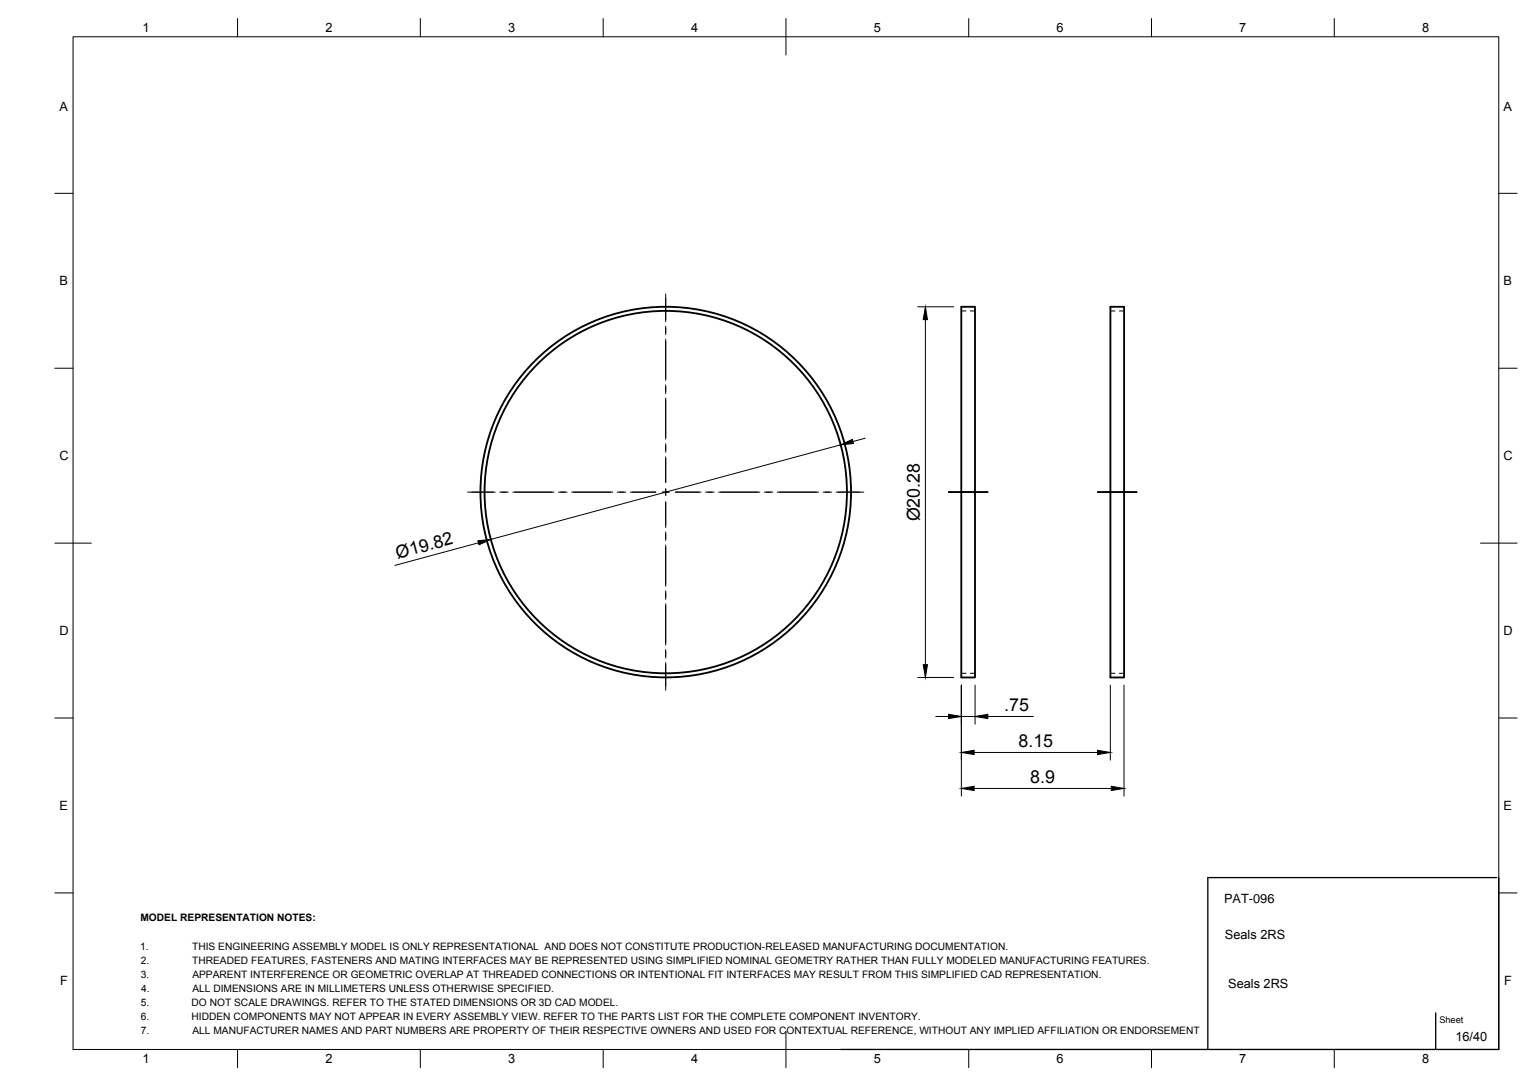
ISO-10303-21;
HEADER;
/* Generated by software containing ST-Developer
 * from STEP Tools, Inc. (www.steptools.com) 
 */

FILE_DESCRIPTION(
/* description */ ('PAT-096'),
/* implementation_level */ '2;1');

FILE_NAME(
/* name */ 'Seals 2RS.step',
/* time_stamp */ '2026-10-29T17:03:14-07:00',
/* author */ (''),
/* organization */ (''),
/* preprocessor_version */ 'ST-DEVELOPER v20.2',
/* originating_system */ 'Autodesk Translation Framework v15.17.0.0',
/* authorisation */ '');

FILE_SCHEMA (('AUTOMOTIVE_DESIGN { 1 0 10303 214 3 1 1 }'));
ENDSEC;

DATA;
#10=MECHANICAL_DESIGN_GEOMETRIC_PRESENTATION_REPRESENTATION('',(#413,#414),#10650);
#344=SHAPE_REPRESENTATION_RELATIONSHIP('SRR','None',#10805,#375);
#375=ADVANCED_BREP_SHAPE_REPRESENTATION('',(#451,#452),#10623);
#413=STYLED_ITEM('',(#11064),#451);
#414=STYLED_ITEM('',(#11064),#452);
#451=MANIFOLD_SOLID_BREP('Body1',#5547);
#452=MANIFOLD_SOLID_BREP('Body2',#5548);
#528=FACE_BOUND('',#1302,.T.);
#529=FACE_BOUND('',#1305,.T.);
#530=FACE_BOUND('',#1308,.T.);
#531=FACE_BOUND('',#1311,.T.);
#661=PLANE('',#6196);
#662=PLANE('',#6201);
#663=PLANE('',#6204);
#664=PLANE('',#6209);
#910=FACE_OUTER_BOUND('',#1301,.T.);
#911=FACE_OUTER_BOUND('',#1303,.T.);
#912=FACE_OUTER_BOUND('',#1304,.T.);
#913=FACE_OUTER_BOUND('',#1306,.T.);
#914=FACE_OUTER_BOUND('',#1307,.T.);
#915=FACE_OUTER_BOUND('',#1309,.T.);
#916=FACE_OUTER_BOUND('',#1310,.T.);
#917=FACE_OUTER_BOUND('',#1312,.T.);
#1301=EDGE_LOOP('',(#4231));
#1302=EDGE_LOOP('',(#4232));
#1303=EDGE_LOOP('',(#4233,#4234,#4235,#4236));
#1304=EDGE_LOOP('',(#4237));
#1305=EDGE_LOOP('',(#4238));
#1306=EDGE_LOOP('',(#4239,#4240,#4241,#4242));
#1307=EDGE_LOOP('',(#4243));
#1308=EDGE_LOOP('',(#4244));
#1309=EDGE_LOOP('',(#4245,#4246,#4247,#4248));
#1310=EDGE_LOOP('',(#4249));
#1311=EDGE_LOOP('',(#4250));
#1312=EDGE_LOOP('',(#4251,#4252,#4253,#4254));
#1688=LINE('',#9497,#2017);
#1689=LINE('',#9502,#2018);
#1690=LINE('',#9511,#2019);
#1691=LINE('',#9516,#2020);
#2017=VECTOR('',#7330,1.013815);
#2018=VECTOR('',#7337,0.991185);
#2019=VECTOR('',#7348,1.013815);
#2020=VECTOR('',#7355,0.991185);
#2408=CIRCLE('',#6197,1.013815);
#2409=CIRCLE('',#6198,0.991185);
#2410=CIRCLE('',#6200,1.013815);
#2411=CIRCLE('',#6202,0.991185);
#2412=CIRCLE('',#6205,1.013815);
#2413=CIRCLE('',#6206,0.991185);
#2414=CIRCLE('',#6208,1.013815);
#2415=CIRCLE('',#6210,0.991185);
#2759=VERTEX_POINT('',#9490);
#2760=VERTEX_POINT('',#9492);
#2761=VERTEX_POINT('',#9495);
#2762=VERTEX_POINT('',#9499);
#2763=VERTEX_POINT('',#9504);
#2764=VERTEX_POINT('',#9506);
#2765=VERTEX_POINT('',#9509);
#2766=VERTEX_POINT('',#9513);
#3294=EDGE_CURVE('',#2759,#2759,#2408,.T.);
#3295=EDGE_CURVE('',#2760,#2760,#2409,.T.);
#3296=EDGE_CURVE('',#2761,#2761,#2410,.T.);
#3297=EDGE_CURVE('',#2761,#2759,#1688,.T.);
#3298=EDGE_CURVE('',#2762,#2762,#2411,.T.);
#3299=EDGE_CURVE('',#2762,#2760,#1689,.T.);
#3300=EDGE_CURVE('',#2763,#2763,#2412,.T.);
#3301=EDGE_CURVE('',#2764,#2764,#2413,.T.);
#3302=EDGE_CURVE('',#2765,#2765,#2414,.T.);
#3303=EDGE_CURVE('',#2765,#2763,#1690,.T.);
#3304=EDGE_CURVE('',#2766,#2766,#2415,.T.);
#3305=EDGE_CURVE('',#2766,#2764,#1691,.T.);
#4231=ORIENTED_EDGE('',*,*,#3294,.F.);
#4232=ORIENTED_EDGE('',*,*,#3295,.T.);
#4233=ORIENTED_EDGE('',*,*,#3296,.F.);
#4234=ORIENTED_EDGE('',*,*,#3297,.T.);
#4235=ORIENTED_EDGE('',*,*,#3294,.T.);
#4236=ORIENTED_EDGE('',*,*,#3297,.F.);
#4237=ORIENTED_EDGE('',*,*,#3296,.T.);
#4238=ORIENTED_EDGE('',*,*,#3298,.F.);
#4239=ORIENTED_EDGE('',*,*,#3298,.T.);
#4240=ORIENTED_EDGE('',*,*,#3299,.T.);
#4241=ORIENTED_EDGE('',*,*,#3295,.F.);
#4242=ORIENTED_EDGE('',*,*,#3299,.F.);
#4243=ORIENTED_EDGE('',*,*,#3300,.F.);
#4244=ORIENTED_EDGE('',*,*,#3301,.T.);
#4245=ORIENTED_EDGE('',*,*,#3302,.F.);
#4246=ORIENTED_EDGE('',*,*,#3303,.T.);
#4247=ORIENTED_EDGE('',*,*,#3300,.T.);
#4248=ORIENTED_EDGE('',*,*,#3303,.F.);
#4249=ORIENTED_EDGE('',*,*,#3302,.T.);
#4250=ORIENTED_EDGE('',*,*,#3304,.F.);
#4251=ORIENTED_EDGE('',*,*,#3304,.T.);
#4252=ORIENTED_EDGE('',*,*,#3305,.T.);
#4253=ORIENTED_EDGE('',*,*,#3301,.F.);
#4254=ORIENTED_EDGE('',*,*,#3305,.F.);
#5119=CYLINDRICAL_SURFACE('',#6199,1.013815);
#5120=CYLINDRICAL_SURFACE('',#6203,0.991185);
#5121=CYLINDRICAL_SURFACE('',#6207,1.013815);
#5122=CYLINDRICAL_SURFACE('',#6211,0.991185);
#5315=ADVANCED_FACE('',(#910,#528),#661,.T.);
#5316=ADVANCED_FACE('',(#911),#5119,.T.);
#5317=ADVANCED_FACE('',(#912,#529),#662,.T.);
#5318=ADVANCED_FACE('',(#913),#5120,.F.);
#5319=ADVANCED_FACE('',(#914,#530),#663,.T.);
#5320=ADVANCED_FACE('',(#915),#5121,.T.);
#5321=ADVANCED_FACE('',(#916,#531),#664,.T.);
#5322=ADVANCED_FACE('',(#917),#5122,.F.);
#5547=CLOSED_SHELL('',(#5315,#5316,#5317,#5318));
#5548=CLOSED_SHELL('',(#5319,#5320,#5321,#5322));
#6195=AXIS2_PLACEMENT_3D('',#9488,#7318,#7319);
#6196=AXIS2_PLACEMENT_3D('',#9489,#7320,#7321);
#6197=AXIS2_PLACEMENT_3D('',#9491,#7322,#7323);
#6198=AXIS2_PLACEMENT_3D('',#9493,#7324,#7325);
#6199=AXIS2_PLACEMENT_3D('',#9494,#7326,#7327);
#6200=AXIS2_PLACEMENT_3D('',#9496,#7328,#7329);
#6201=AXIS2_PLACEMENT_3D('',#9498,#7331,#7332);
#6202=AXIS2_PLACEMENT_3D('',#9500,#7333,#7334);
#6203=AXIS2_PLACEMENT_3D('',#9501,#7335,#7336);
#6204=AXIS2_PLACEMENT_3D('',#9503,#7338,#7339);
#6205=AXIS2_PLACEMENT_3D('',#9505,#7340,#7341);
#6206=AXIS2_PLACEMENT_3D('',#9507,#7342,#7343);
#6207=AXIS2_PLACEMENT_3D('',#9508,#7344,#7345);
#6208=AXIS2_PLACEMENT_3D('',#9510,#7346,#7347);
#6209=AXIS2_PLACEMENT_3D('',#9512,#7349,#7350);
#6210=AXIS2_PLACEMENT_3D('',#9514,#7351,#7352);
#6211=AXIS2_PLACEMENT_3D('',#9515,#7353,#7354);
#7318=DIRECTION('axis',(0.,0.,1.));
#7319=DIRECTION('refdir',(1.,0.,0.));
#7320=DIRECTION('center_axis',(0.,1.,0.));
#7321=DIRECTION('ref_axis',(0.,0.,1.));
#7322=DIRECTION('center_axis',(0.,-1.,0.));
#7323=DIRECTION('ref_axis',(1.,0.,0.));
#7324=DIRECTION('center_axis',(0.,-1.,0.));
#7325=DIRECTION('ref_axis',(1.,0.,0.));
#7326=DIRECTION('center_axis',(0.,-1.,0.));
#7327=DIRECTION('ref_axis',(1.,0.,0.));
#7328=DIRECTION('center_axis',(0.,-1.,0.));
#7329=DIRECTION('ref_axis',(1.,0.,0.));
#7330=DIRECTION('',(0.,1.,0.));
#7331=DIRECTION('center_axis',(0.,-1.,0.));
#7332=DIRECTION('ref_axis',(0.,0.,-1.));
#7333=DIRECTION('center_axis',(0.,-1.,0.));
#7334=DIRECTION('ref_axis',(1.,0.,0.));
#7335=DIRECTION('center_axis',(0.,-1.,0.));
#7336=DIRECTION('ref_axis',(1.,0.,0.));
#7337=DIRECTION('',(0.,1.,0.));
#7338=DIRECTION('center_axis',(0.,1.,0.));
#7339=DIRECTION('ref_axis',(0.,0.,1.));
#7340=DIRECTION('center_axis',(0.,-1.,0.));
#7341=DIRECTION('ref_axis',(1.,0.,0.));
#7342=DIRECTION('center_axis',(0.,-1.,0.));
#7343=DIRECTION('ref_axis',(1.,0.,0.));
#7344=DIRECTION('center_axis',(0.,-1.,0.));
#7345=DIRECTION('ref_axis',(1.,0.,0.));
#7346=DIRECTION('center_axis',(0.,-1.,0.));
#7347=DIRECTION('ref_axis',(1.,0.,0.));
#7348=DIRECTION('',(0.,1.,0.));
#7349=DIRECTION('center_axis',(0.,-1.,0.));
#7350=DIRECTION('ref_axis',(0.,0.,-1.));
#7351=DIRECTION('center_axis',(0.,-1.,0.));
#7352=DIRECTION('ref_axis',(1.,0.,0.));
#7353=DIRECTION('center_axis',(0.,-1.,0.));
#7354=DIRECTION('ref_axis',(1.,0.,0.));
#7355=DIRECTION('',(0.,1.,0.));
#9488=CARTESIAN_POINT('',(0.,0.,0.));
#9489=CARTESIAN_POINT('Origin',(1.013815,0.445,0.));
#9490=CARTESIAN_POINT('',(-1.013815,0.445,-1.24156529467757E-16));
#9491=CARTESIAN_POINT('Origin',(0.,0.445,0.));
#9492=CARTESIAN_POINT('',(-0.991185,0.445,-1.21385153761287E-16));
#9493=CARTESIAN_POINT('Origin',(0.,0.445,0.));
#9494=CARTESIAN_POINT('Origin',(0.,0.4075,0.));
#9495=CARTESIAN_POINT('',(-1.013815,0.37,-1.24156529467757E-16));
#9496=CARTESIAN_POINT('Origin',(0.,0.37,0.));
#9497=CARTESIAN_POINT('',(-1.013815,0.4075,-1.24156529467757E-16));
#9498=CARTESIAN_POINT('Origin',(0.991185,0.37,0.));
#9499=CARTESIAN_POINT('',(-0.991185,0.37,-1.21385153761287E-16));
#9500=CARTESIAN_POINT('Origin',(0.,0.37,0.));
#9501=CARTESIAN_POINT('Origin',(0.,0.4075,0.));
#9502=CARTESIAN_POINT('',(-0.991185,0.4075,-1.21385153761287E-16));
#9503=CARTESIAN_POINT('Origin',(1.013815,-0.37,0.));
#9504=CARTESIAN_POINT('',(-1.013815,-0.37,-1.24156529467757E-16));
#9505=CARTESIAN_POINT('Origin',(0.,-0.37,0.));
#9506=CARTESIAN_POINT('',(-0.991185,-0.37,-1.21385153761287E-16));
#9507=CARTESIAN_POINT('Origin',(0.,-0.37,0.));
#9508=CARTESIAN_POINT('Origin',(0.,-0.4075,0.));
#9509=CARTESIAN_POINT('',(-1.013815,-0.445,-1.24156529467757E-16));
#9510=CARTESIAN_POINT('Origin',(0.,-0.445,0.));
#9511=CARTESIAN_POINT('',(-1.013815,-0.4075,-1.24156529467757E-16));
#9512=CARTESIAN_POINT('Origin',(0.991185,-0.445,0.));
#9513=CARTESIAN_POINT('',(-0.991185,-0.445,-1.21385153761287E-16));
#9514=CARTESIAN_POINT('Origin',(0.,-0.445,0.));
#9515=CARTESIAN_POINT('Origin',(0.,-0.4075,0.));
#9516=CARTESIAN_POINT('',(-0.991185,-0.4075,-1.21385153761287E-16));
#10584=UNCERTAINTY_MEASURE_WITH_UNIT(LENGTH_MEASURE(0.001),#10651,
'DISTANCE_ACCURACY_VALUE',
'Maximum model space distance between geometric entities at asserted c
onnectivities');
#10611=UNCERTAINTY_MEASURE_WITH_UNIT(LENGTH_MEASURE(0.001),#10651,
'DISTANCE_ACCURACY_VALUE',
'Maximum model space distance between geometric entities at asserted c
onnectivities');
#10623=(
GEOMETRIC_REPRESENTATION_CONTEXT(3)
GLOBAL_UNCERTAINTY_ASSIGNED_CONTEXT((#10584))
GLOBAL_UNIT_ASSIGNED_CONTEXT((#10651,#10653,#10654))
REPRESENTATION_CONTEXT('','3D')
);
#10650=(
GEOMETRIC_REPRESENTATION_CONTEXT(3)
GLOBAL_UNCERTAINTY_ASSIGNED_CONTEXT((#10611))
GLOBAL_UNIT_ASSIGNED_CONTEXT((#10651,#10653,#10654))
REPRESENTATION_CONTEXT('','3D')
);
#10651=(
LENGTH_UNIT()
NAMED_UNIT(*)
SI_UNIT(.CENTI.,.METRE.)
);
#10653=(
NAMED_UNIT(*)
PLANE_ANGLE_UNIT()
SI_UNIT($,.RADIAN.)
);
#10654=(
NAMED_UNIT(*)
SI_UNIT($,.STERADIAN.)
SOLID_ANGLE_UNIT()
);
#10666=SHAPE_DEFINITION_REPRESENTATION(#10704,#10805);
#10704=PRODUCT_DEFINITION_SHAPE('',$,#10844);
#10805=SHAPE_REPRESENTATION('',(#6195),#10623);
#10832=PRODUCT_DEFINITION_CONTEXT('part definition',#10948,'design');
#10844=PRODUCT_DEFINITION('Seals 2RS','Seals 2RS',#10882,#10832);
#10882=PRODUCT_DEFINITION_FORMATION('',$,#10961);
#10948=APPLICATION_CONTEXT(
'Core Data for Automotive Mechanical Design Process');
#10949=PRODUCT_CONTEXT('part definition',#10948,'mechanical');
#10961=PRODUCT('Seals 2RS','Seals 2RS','Seals 2RS',(#10949));
#11058=COLOUR_RGB('Grey',0.48,0.52,0.57);
#11059=FILL_AREA_STYLE_COLOUR('',#11058);
#11060=FILL_AREA_STYLE('',(#11059));
#11061=SURFACE_STYLE_FILL_AREA(#11060);
#11062=SURFACE_SIDE_STYLE('',(#11061));
#11063=SURFACE_STYLE_USAGE(.BOTH.,#11062);
#11064=PRESENTATION_STYLE_ASSIGNMENT((#11063));
ENDSEC;
END-ISO-10303-21;
